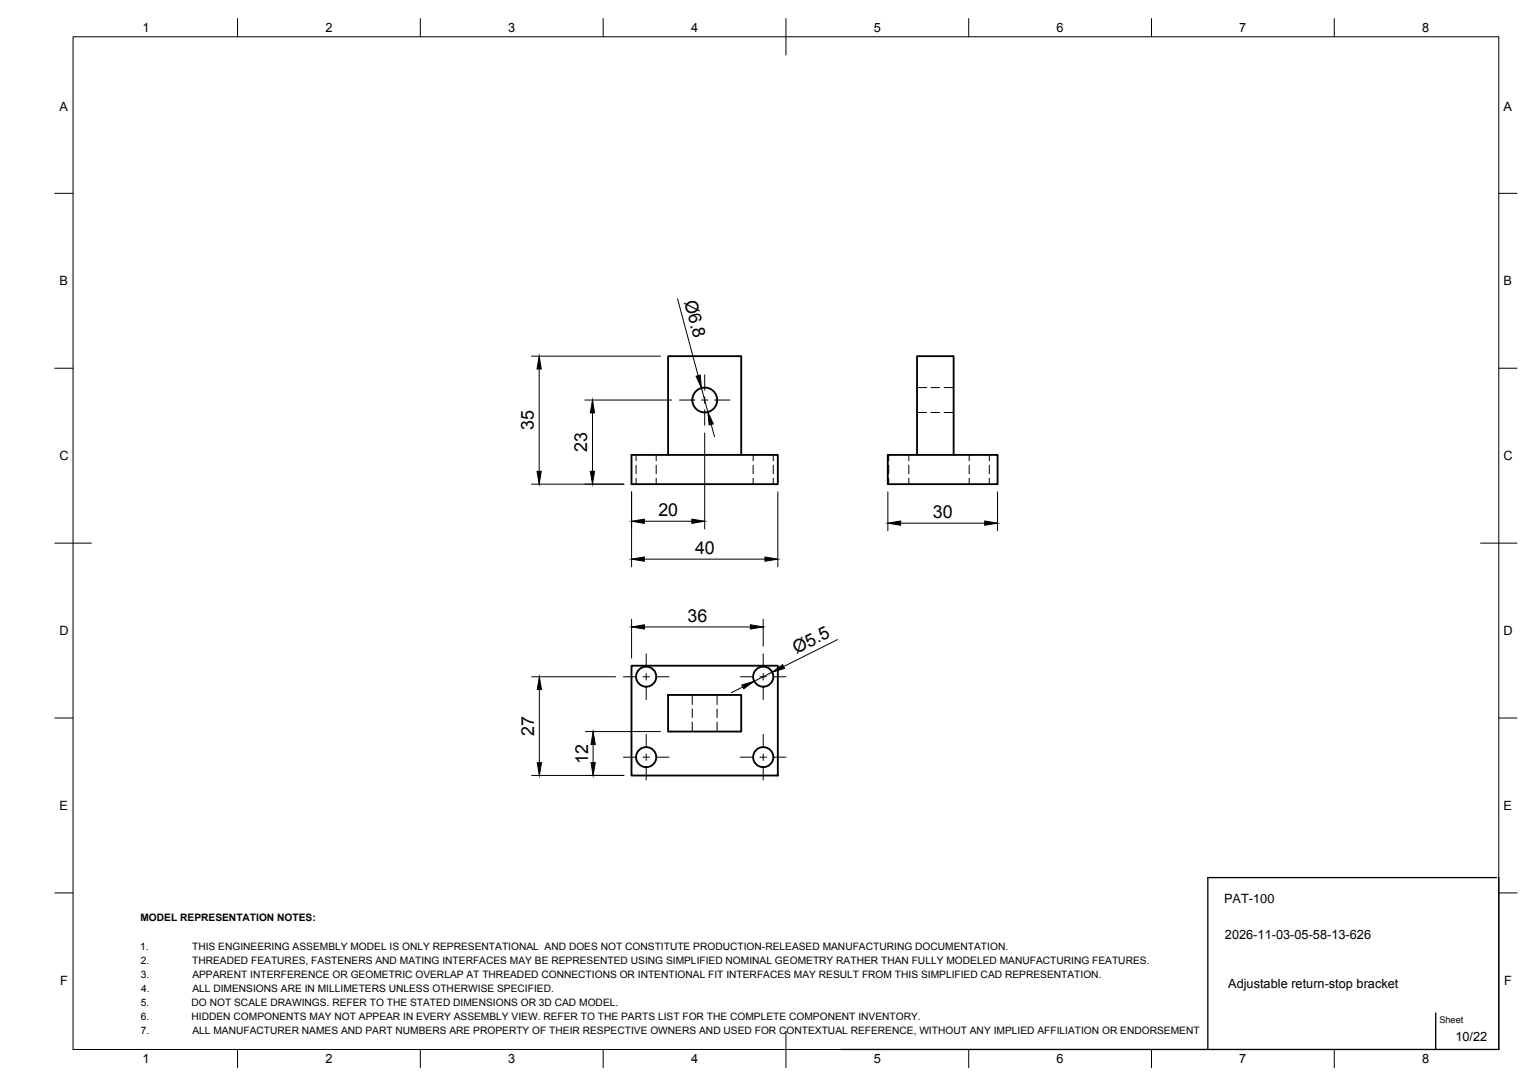
ISO-10303-21;
HEADER;
/* Generated by software containing ST-Developer
 * from STEP Tools, Inc. (www.steptools.com) 
 */

FILE_DESCRIPTION(
/* description */ (''),
/* implementation_level */ '2;1');

FILE_NAME(
/* name */ 'Adjustable return-stop bracket.step',
/* time_stamp */ '2026-10-29T16:43:51-07:00',
/* author */ (''),
/* organization */ (''),
/* preprocessor_version */ 'ST-DEVELOPER v20.2',
/* originating_system */ 'Autodesk Translation Framework v15.17.0.0',
/* authorisation */ '');

FILE_SCHEMA (('AUTOMOTIVE_DESIGN { 1 0 10303 214 3 1 1 }'));
ENDSEC;

DATA;
#10=MECHANICAL_DESIGN_GEOMETRIC_PRESENTATION_REPRESENTATION('',(#371),#10292);
#325=SHAPE_REPRESENTATION_RELATIONSHIP('SRR','None',#10421,#348);
#348=ADVANCED_BREP_SHAPE_REPRESENTATION('',(#393),#10273);
#371=STYLED_ITEM('',(#10607),#393);
#393=MANIFOLD_SOLID_BREP('Body1',#5014);
#455=FACE_BOUND('',#1140,.T.);
#456=FACE_BOUND('',#1142,.T.);
#457=FACE_BOUND('',#1148,.T.);
#458=FACE_BOUND('',#1149,.T.);
#459=FACE_BOUND('',#1150,.T.);
#460=FACE_BOUND('',#1151,.T.);
#461=FACE_BOUND('',#1152,.T.);
#462=FACE_BOUND('',#1154,.T.);
#463=FACE_BOUND('',#1155,.T.);
#464=FACE_BOUND('',#1156,.T.);
#465=FACE_BOUND('',#1157,.T.);
#580=PLANE('',#5462);
#581=PLANE('',#5463);
#582=PLANE('',#5464);
#583=PLANE('',#5465);
#584=PLANE('',#5466);
#585=PLANE('',#5467);
#586=PLANE('',#5468);
#587=PLANE('',#5469);
#588=PLANE('',#5470);
#589=PLANE('',#5471);
#590=PLANE('',#5472);
#794=FACE_OUTER_BOUND('',#1131,.T.);
#795=FACE_OUTER_BOUND('',#1132,.T.);
#796=FACE_OUTER_BOUND('',#1133,.T.);
#797=FACE_OUTER_BOUND('',#1134,.T.);
#798=FACE_OUTER_BOUND('',#1135,.T.);
#799=FACE_OUTER_BOUND('',#1136,.T.);
#800=FACE_OUTER_BOUND('',#1137,.T.);
#801=FACE_OUTER_BOUND('',#1138,.T.);
#802=FACE_OUTER_BOUND('',#1139,.T.);
#803=FACE_OUTER_BOUND('',#1141,.T.);
#804=FACE_OUTER_BOUND('',#1143,.T.);
#805=FACE_OUTER_BOUND('',#1144,.T.);
#806=FACE_OUTER_BOUND('',#1145,.T.);
#807=FACE_OUTER_BOUND('',#1146,.T.);
#808=FACE_OUTER_BOUND('',#1147,.T.);
#809=FACE_OUTER_BOUND('',#1153,.T.);
#1131=EDGE_LOOP('',(#3801,#3802,#3803,#3804));
#1132=EDGE_LOOP('',(#3805,#3806,#3807,#3808));
#1133=EDGE_LOOP('',(#3809,#3810,#3811,#3812));
#1134=EDGE_LOOP('',(#3813,#3814,#3815,#3816));
#1135=EDGE_LOOP('',(#3817,#3818,#3819,#3820));
#1136=EDGE_LOOP('',(#3821,#3822,#3823,#3824));
#1137=EDGE_LOOP('',(#3825,#3826,#3827,#3828));
#1138=EDGE_LOOP('',(#3829,#3830,#3831,#3832));
#1139=EDGE_LOOP('',(#3833,#3834,#3835,#3836));
#1140=EDGE_LOOP('',(#3837));
#1141=EDGE_LOOP('',(#3838,#3839,#3840,#3841));
#1142=EDGE_LOOP('',(#3842));
#1143=EDGE_LOOP('',(#3843,#3844,#3845,#3846));
#1144=EDGE_LOOP('',(#3847,#3848,#3849,#3850));
#1145=EDGE_LOOP('',(#3851,#3852,#3853,#3854));
#1146=EDGE_LOOP('',(#3855,#3856,#3857,#3858));
#1147=EDGE_LOOP('',(#3859,#3860,#3861,#3862));
#1148=EDGE_LOOP('',(#3863,#3864,#3865,#3866));
#1149=EDGE_LOOP('',(#3867));
#1150=EDGE_LOOP('',(#3868));
#1151=EDGE_LOOP('',(#3869));
#1152=EDGE_LOOP('',(#3870));
#1153=EDGE_LOOP('',(#3871,#3872,#3873,#3874));
#1154=EDGE_LOOP('',(#3875));
#1155=EDGE_LOOP('',(#3876));
#1156=EDGE_LOOP('',(#3877));
#1157=EDGE_LOOP('',(#3878));
#1542=LINE('',#7828,#1934);
#1543=LINE('',#7834,#1935);
#1544=LINE('',#7840,#1936);
#1545=LINE('',#7846,#1937);
#1546=LINE('',#7852,#1938);
#1547=LINE('',#7857,#1939);
#1548=LINE('',#7859,#1940);
#1549=LINE('',#7861,#1941);
#1550=LINE('',#7862,#1942);
#1551=LINE('',#7865,#1943);
#1552=LINE('',#7867,#1944);
#1553=LINE('',#7868,#1945);
#1554=LINE('',#7871,#1946);
#1555=LINE('',#7873,#1947);
#1556=LINE('',#7874,#1948);
#1557=LINE('',#7876,#1949);
#1558=LINE('',#7878,#1950);
#1559=LINE('',#7882,#1951);
#1560=LINE('',#7884,#1952);
#1561=LINE('',#7886,#1953);
#1562=LINE('',#7887,#1954);
#1563=LINE('',#7890,#1955);
#1564=LINE('',#7892,#1956);
#1565=LINE('',#7893,#1957);
#1566=LINE('',#7896,#1958);
#1567=LINE('',#7898,#1959);
#1568=LINE('',#7899,#1960);
#1569=LINE('',#7901,#1961);
#1570=LINE('',#7902,#1962);
#1934=VECTOR('',#6315,0.34);
#1935=VECTOR('',#6322,0.275);
#1936=VECTOR('',#6329,0.275);
#1937=VECTOR('',#6336,0.275);
#1938=VECTOR('',#6343,0.275);
#1939=VECTOR('',#6348,1.);
#1940=VECTOR('',#6349,1.);
#1941=VECTOR('',#6350,1.);
#1942=VECTOR('',#6351,1.);
#1943=VECTOR('',#6354,1.);
#1944=VECTOR('',#6355,1.);
#1945=VECTOR('',#6356,1.);
#1946=VECTOR('',#6359,1.);
#1947=VECTOR('',#6360,1.);
#1948=VECTOR('',#6361,1.);
#1949=VECTOR('',#6364,1.);
#1950=VECTOR('',#6367,1.);
#1951=VECTOR('',#6370,1.);
#1952=VECTOR('',#6371,1.);
#1953=VECTOR('',#6372,1.);
#1954=VECTOR('',#6373,1.);
#1955=VECTOR('',#6376,1.);
#1956=VECTOR('',#6377,1.);
#1957=VECTOR('',#6378,1.);
#1958=VECTOR('',#6381,1.);
#1959=VECTOR('',#6382,1.);
#1960=VECTOR('',#6383,1.);
#1961=VECTOR('',#6386,1.);
#1962=VECTOR('',#6387,1.);
#2260=CIRCLE('',#5448,0.34);
#2261=CIRCLE('',#5449,0.34);
#2262=CIRCLE('',#5451,0.275);
#2263=CIRCLE('',#5452,0.275);
#2264=CIRCLE('',#5454,0.275);
#2265=CIRCLE('',#5455,0.275);
#2266=CIRCLE('',#5457,0.275);
#2267=CIRCLE('',#5458,0.275);
#2268=CIRCLE('',#5460,0.275);
#2269=CIRCLE('',#5461,0.275);
#2523=VERTEX_POINT('',#7825);
#2524=VERTEX_POINT('',#7827);
#2525=VERTEX_POINT('',#7831);
#2526=VERTEX_POINT('',#7833);
#2527=VERTEX_POINT('',#7837);
#2528=VERTEX_POINT('',#7839);
#2529=VERTEX_POINT('',#7843);
#2530=VERTEX_POINT('',#7845);
#2531=VERTEX_POINT('',#7849);
#2532=VERTEX_POINT('',#7851);
#2533=VERTEX_POINT('',#7855);
#2534=VERTEX_POINT('',#7856);
#2535=VERTEX_POINT('',#7858);
#2536=VERTEX_POINT('',#7860);
#2537=VERTEX_POINT('',#7864);
#2538=VERTEX_POINT('',#7866);
#2539=VERTEX_POINT('',#7870);
#2540=VERTEX_POINT('',#7872);
#2541=VERTEX_POINT('',#7880);
#2542=VERTEX_POINT('',#7881);
#2543=VERTEX_POINT('',#7883);
#2544=VERTEX_POINT('',#7885);
#2545=VERTEX_POINT('',#7889);
#2546=VERTEX_POINT('',#7891);
#2547=VERTEX_POINT('',#7895);
#2548=VERTEX_POINT('',#7897);
#2991=EDGE_CURVE('',#2523,#2523,#2260,.T.);
#2992=EDGE_CURVE('',#2523,#2524,#1542,.T.);
#2993=EDGE_CURVE('',#2524,#2524,#2261,.T.);
#2994=EDGE_CURVE('',#2525,#2525,#2262,.T.);
#2995=EDGE_CURVE('',#2525,#2526,#1543,.T.);
#2996=EDGE_CURVE('',#2526,#2526,#2263,.T.);
#2997=EDGE_CURVE('',#2527,#2527,#2264,.T.);
#2998=EDGE_CURVE('',#2527,#2528,#1544,.T.);
#2999=EDGE_CURVE('',#2528,#2528,#2265,.T.);
#3000=EDGE_CURVE('',#2529,#2529,#2266,.T.);
#3001=EDGE_CURVE('',#2529,#2530,#1545,.T.);
#3002=EDGE_CURVE('',#2530,#2530,#2267,.T.);
#3003=EDGE_CURVE('',#2531,#2531,#2268,.T.);
#3004=EDGE_CURVE('',#2531,#2532,#1546,.T.);
#3005=EDGE_CURVE('',#2532,#2532,#2269,.T.);
#3006=EDGE_CURVE('',#2533,#2534,#1547,.T.);
#3007=EDGE_CURVE('',#2534,#2535,#1548,.T.);
#3008=EDGE_CURVE('',#2536,#2535,#1549,.T.);
#3009=EDGE_CURVE('',#2533,#2536,#1550,.T.);
#3010=EDGE_CURVE('',#2537,#2533,#1551,.T.);
#3011=EDGE_CURVE('',#2538,#2536,#1552,.T.);
#3012=EDGE_CURVE('',#2537,#2538,#1553,.T.);
#3013=EDGE_CURVE('',#2534,#2539,#1554,.T.);
#3014=EDGE_CURVE('',#2540,#2539,#1555,.T.);
#3015=EDGE_CURVE('',#2535,#2540,#1556,.T.);
#3016=EDGE_CURVE('',#2538,#2540,#1557,.T.);
#3017=EDGE_CURVE('',#2539,#2537,#1558,.T.);
#3018=EDGE_CURVE('',#2541,#2542,#1559,.T.);
#3019=EDGE_CURVE('',#2542,#2543,#1560,.T.);
#3020=EDGE_CURVE('',#2544,#2543,#1561,.T.);
#3021=EDGE_CURVE('',#2541,#2544,#1562,.T.);
#3022=EDGE_CURVE('',#2545,#2541,#1563,.T.);
#3023=EDGE_CURVE('',#2546,#2544,#1564,.T.);
#3024=EDGE_CURVE('',#2545,#2546,#1565,.T.);
#3025=EDGE_CURVE('',#2547,#2545,#1566,.T.);
#3026=EDGE_CURVE('',#2548,#2546,#1567,.T.);
#3027=EDGE_CURVE('',#2547,#2548,#1568,.T.);
#3028=EDGE_CURVE('',#2542,#2547,#1569,.T.);
#3029=EDGE_CURVE('',#2543,#2548,#1570,.T.);
#3801=ORIENTED_EDGE('',*,*,#2991,.F.);
#3802=ORIENTED_EDGE('',*,*,#2992,.T.);
#3803=ORIENTED_EDGE('',*,*,#2993,.F.);
#3804=ORIENTED_EDGE('',*,*,#2992,.F.);
#3805=ORIENTED_EDGE('',*,*,#2994,.F.);
#3806=ORIENTED_EDGE('',*,*,#2995,.T.);
#3807=ORIENTED_EDGE('',*,*,#2996,.F.);
#3808=ORIENTED_EDGE('',*,*,#2995,.F.);
#3809=ORIENTED_EDGE('',*,*,#2997,.F.);
#3810=ORIENTED_EDGE('',*,*,#2998,.T.);
#3811=ORIENTED_EDGE('',*,*,#2999,.F.);
#3812=ORIENTED_EDGE('',*,*,#2998,.F.);
#3813=ORIENTED_EDGE('',*,*,#3000,.F.);
#3814=ORIENTED_EDGE('',*,*,#3001,.T.);
#3815=ORIENTED_EDGE('',*,*,#3002,.F.);
#3816=ORIENTED_EDGE('',*,*,#3001,.F.);
#3817=ORIENTED_EDGE('',*,*,#3003,.F.);
#3818=ORIENTED_EDGE('',*,*,#3004,.T.);
#3819=ORIENTED_EDGE('',*,*,#3005,.F.);
#3820=ORIENTED_EDGE('',*,*,#3004,.F.);
#3821=ORIENTED_EDGE('',*,*,#3006,.T.);
#3822=ORIENTED_EDGE('',*,*,#3007,.T.);
#3823=ORIENTED_EDGE('',*,*,#3008,.F.);
#3824=ORIENTED_EDGE('',*,*,#3009,.F.);
#3825=ORIENTED_EDGE('',*,*,#3010,.T.);
#3826=ORIENTED_EDGE('',*,*,#3009,.T.);
#3827=ORIENTED_EDGE('',*,*,#3011,.F.);
#3828=ORIENTED_EDGE('',*,*,#3012,.F.);
#3829=ORIENTED_EDGE('',*,*,#3013,.T.);
#3830=ORIENTED_EDGE('',*,*,#3014,.F.);
#3831=ORIENTED_EDGE('',*,*,#3015,.F.);
#3832=ORIENTED_EDGE('',*,*,#3007,.F.);
#3833=ORIENTED_EDGE('',*,*,#3015,.T.);
#3834=ORIENTED_EDGE('',*,*,#3016,.F.);
#3835=ORIENTED_EDGE('',*,*,#3011,.T.);
#3836=ORIENTED_EDGE('',*,*,#3008,.T.);
#3837=ORIENTED_EDGE('',*,*,#2993,.T.);
#3838=ORIENTED_EDGE('',*,*,#3013,.F.);
#3839=ORIENTED_EDGE('',*,*,#3006,.F.);
#3840=ORIENTED_EDGE('',*,*,#3010,.F.);
#3841=ORIENTED_EDGE('',*,*,#3017,.F.);
#3842=ORIENTED_EDGE('',*,*,#2991,.T.);
#3843=ORIENTED_EDGE('',*,*,#3018,.T.);
#3844=ORIENTED_EDGE('',*,*,#3019,.T.);
#3845=ORIENTED_EDGE('',*,*,#3020,.F.);
#3846=ORIENTED_EDGE('',*,*,#3021,.F.);
#3847=ORIENTED_EDGE('',*,*,#3022,.T.);
#3848=ORIENTED_EDGE('',*,*,#3021,.T.);
#3849=ORIENTED_EDGE('',*,*,#3023,.F.);
#3850=ORIENTED_EDGE('',*,*,#3024,.F.);
#3851=ORIENTED_EDGE('',*,*,#3025,.T.);
#3852=ORIENTED_EDGE('',*,*,#3024,.T.);
#3853=ORIENTED_EDGE('',*,*,#3026,.F.);
#3854=ORIENTED_EDGE('',*,*,#3027,.F.);
#3855=ORIENTED_EDGE('',*,*,#3028,.T.);
#3856=ORIENTED_EDGE('',*,*,#3027,.T.);
#3857=ORIENTED_EDGE('',*,*,#3029,.F.);
#3858=ORIENTED_EDGE('',*,*,#3019,.F.);
#3859=ORIENTED_EDGE('',*,*,#3029,.T.);
#3860=ORIENTED_EDGE('',*,*,#3026,.T.);
#3861=ORIENTED_EDGE('',*,*,#3023,.T.);
#3862=ORIENTED_EDGE('',*,*,#3020,.T.);
#3863=ORIENTED_EDGE('',*,*,#3014,.T.);
#3864=ORIENTED_EDGE('',*,*,#3017,.T.);
#3865=ORIENTED_EDGE('',*,*,#3012,.T.);
#3866=ORIENTED_EDGE('',*,*,#3016,.T.);
#3867=ORIENTED_EDGE('',*,*,#3005,.T.);
#3868=ORIENTED_EDGE('',*,*,#3002,.T.);
#3869=ORIENTED_EDGE('',*,*,#2999,.T.);
#3870=ORIENTED_EDGE('',*,*,#2996,.T.);
#3871=ORIENTED_EDGE('',*,*,#3028,.F.);
#3872=ORIENTED_EDGE('',*,*,#3018,.F.);
#3873=ORIENTED_EDGE('',*,*,#3022,.F.);
#3874=ORIENTED_EDGE('',*,*,#3025,.F.);
#3875=ORIENTED_EDGE('',*,*,#2994,.T.);
#3876=ORIENTED_EDGE('',*,*,#2997,.T.);
#3877=ORIENTED_EDGE('',*,*,#3000,.T.);
#3878=ORIENTED_EDGE('',*,*,#3003,.T.);
#4667=CYLINDRICAL_SURFACE('',#5447,0.34);
#4668=CYLINDRICAL_SURFACE('',#5450,0.275);
#4669=CYLINDRICAL_SURFACE('',#5453,0.275);
#4670=CYLINDRICAL_SURFACE('',#5456,0.275);
#4671=CYLINDRICAL_SURFACE('',#5459,0.275);
#4803=ADVANCED_FACE('',(#794),#4667,.F.);
#4804=ADVANCED_FACE('',(#795),#4668,.F.);
#4805=ADVANCED_FACE('',(#796),#4669,.F.);
#4806=ADVANCED_FACE('',(#797),#4670,.F.);
#4807=ADVANCED_FACE('',(#798),#4671,.F.);
#4808=ADVANCED_FACE('',(#799),#580,.T.);
#4809=ADVANCED_FACE('',(#800),#581,.T.);
#4810=ADVANCED_FACE('',(#801),#582,.T.);
#4811=ADVANCED_FACE('',(#802,#455),#583,.T.);
#4812=ADVANCED_FACE('',(#803,#456),#584,.F.);
#4813=ADVANCED_FACE('',(#804),#585,.T.);
#4814=ADVANCED_FACE('',(#805),#586,.T.);
#4815=ADVANCED_FACE('',(#806),#587,.T.);
#4816=ADVANCED_FACE('',(#807),#588,.T.);
#4817=ADVANCED_FACE('',(#808,#457,#458,#459,#460,#461),#589,.T.);
#4818=ADVANCED_FACE('',(#809,#462,#463,#464,#465),#590,.F.);
#5014=CLOSED_SHELL('',(#4803,#4804,#4805,#4806,#4807,#4808,#4809,#4810,
#4811,#4812,#4813,#4814,#4815,#4816,#4817,#4818));
#5446=AXIS2_PLACEMENT_3D('',#7823,#6309,#6310);
#5447=AXIS2_PLACEMENT_3D('',#7824,#6311,#6312);
#5448=AXIS2_PLACEMENT_3D('',#7826,#6313,#6314);
#5449=AXIS2_PLACEMENT_3D('',#7829,#6316,#6317);
#5450=AXIS2_PLACEMENT_3D('',#7830,#6318,#6319);
#5451=AXIS2_PLACEMENT_3D('',#7832,#6320,#6321);
#5452=AXIS2_PLACEMENT_3D('',#7835,#6323,#6324);
#5453=AXIS2_PLACEMENT_3D('',#7836,#6325,#6326);
#5454=AXIS2_PLACEMENT_3D('',#7838,#6327,#6328);
#5455=AXIS2_PLACEMENT_3D('',#7841,#6330,#6331);
#5456=AXIS2_PLACEMENT_3D('',#7842,#6332,#6333);
#5457=AXIS2_PLACEMENT_3D('',#7844,#6334,#6335);
#5458=AXIS2_PLACEMENT_3D('',#7847,#6337,#6338);
#5459=AXIS2_PLACEMENT_3D('',#7848,#6339,#6340);
#5460=AXIS2_PLACEMENT_3D('',#7850,#6341,#6342);
#5461=AXIS2_PLACEMENT_3D('',#7853,#6344,#6345);
#5462=AXIS2_PLACEMENT_3D('',#7854,#6346,#6347);
#5463=AXIS2_PLACEMENT_3D('',#7863,#6352,#6353);
#5464=AXIS2_PLACEMENT_3D('',#7869,#6357,#6358);
#5465=AXIS2_PLACEMENT_3D('',#7875,#6362,#6363);
#5466=AXIS2_PLACEMENT_3D('',#7877,#6365,#6366);
#5467=AXIS2_PLACEMENT_3D('',#7879,#6368,#6369);
#5468=AXIS2_PLACEMENT_3D('',#7888,#6374,#6375);
#5469=AXIS2_PLACEMENT_3D('',#7894,#6379,#6380);
#5470=AXIS2_PLACEMENT_3D('',#7900,#6384,#6385);
#5471=AXIS2_PLACEMENT_3D('',#7903,#6388,#6389);
#5472=AXIS2_PLACEMENT_3D('',#7904,#6390,#6391);
#6309=DIRECTION('axis',(0.,0.,1.));
#6310=DIRECTION('refdir',(1.,0.,0.));
#6311=DIRECTION('center_axis',(1.,0.,0.));
#6312=DIRECTION('ref_axis',(0.,0.,-1.));
#6313=DIRECTION('center_axis',(1.,0.,0.));
#6314=DIRECTION('ref_axis',(0.,0.,-1.));
#6315=DIRECTION('',(1.,0.,0.));
#6316=DIRECTION('center_axis',(-1.,0.,0.));
#6317=DIRECTION('ref_axis',(0.,0.,-1.));
#6318=DIRECTION('center_axis',(0.,0.,1.));
#6319=DIRECTION('ref_axis',(1.,0.,0.));
#6320=DIRECTION('center_axis',(0.,0.,1.));
#6321=DIRECTION('ref_axis',(1.,0.,0.));
#6322=DIRECTION('',(0.,0.,1.));
#6323=DIRECTION('center_axis',(0.,0.,-1.));
#6324=DIRECTION('ref_axis',(1.,0.,0.));
#6325=DIRECTION('center_axis',(0.,0.,1.));
#6326=DIRECTION('ref_axis',(1.,0.,0.));
#6327=DIRECTION('center_axis',(0.,0.,1.));
#6328=DIRECTION('ref_axis',(1.,0.,0.));
#6329=DIRECTION('',(0.,0.,1.));
#6330=DIRECTION('center_axis',(0.,0.,-1.));
#6331=DIRECTION('ref_axis',(1.,0.,0.));
#6332=DIRECTION('center_axis',(0.,0.,1.));
#6333=DIRECTION('ref_axis',(1.,0.,0.));
#6334=DIRECTION('center_axis',(0.,0.,1.));
#6335=DIRECTION('ref_axis',(1.,0.,0.));
#6336=DIRECTION('',(0.,0.,1.));
#6337=DIRECTION('center_axis',(0.,0.,-1.));
#6338=DIRECTION('ref_axis',(1.,0.,0.));
#6339=DIRECTION('center_axis',(0.,0.,1.));
#6340=DIRECTION('ref_axis',(1.,0.,0.));
#6341=DIRECTION('center_axis',(0.,0.,1.));
#6342=DIRECTION('ref_axis',(1.,0.,0.));
#6343=DIRECTION('',(0.,0.,1.));
#6344=DIRECTION('center_axis',(0.,0.,-1.));
#6345=DIRECTION('ref_axis',(1.,0.,0.));
#6346=DIRECTION('center_axis',(0.,0.,1.));
#6347=DIRECTION('ref_axis',(0.,-1.,0.));
#6348=DIRECTION('',(0.,-1.,0.));
#6349=DIRECTION('',(1.,0.,0.));
#6350=DIRECTION('',(0.,-1.,0.));
#6351=DIRECTION('',(1.,0.,0.));
#6352=DIRECTION('center_axis',(0.,1.,0.));
#6353=DIRECTION('ref_axis',(0.,0.,1.));
#6354=DIRECTION('',(0.,0.,1.));
#6355=DIRECTION('',(0.,0.,1.));
#6356=DIRECTION('',(1.,0.,0.));
#6357=DIRECTION('center_axis',(0.,-1.,0.));
#6358=DIRECTION('ref_axis',(0.,0.,-1.));
#6359=DIRECTION('',(0.,0.,-1.));
#6360=DIRECTION('',(-1.,0.,0.));
#6361=DIRECTION('',(0.,0.,-1.));
#6362=DIRECTION('center_axis',(1.,0.,0.));
#6363=DIRECTION('ref_axis',(0.,0.,-1.));
#6364=DIRECTION('',(0.,-1.,0.));
#6365=DIRECTION('center_axis',(1.,0.,0.));
#6366=DIRECTION('ref_axis',(0.,0.,-1.));
#6367=DIRECTION('',(0.,1.,0.));
#6368=DIRECTION('center_axis',(0.,1.,0.));
#6369=DIRECTION('ref_axis',(-1.,0.,0.));
#6370=DIRECTION('',(-1.,0.,0.));
#6371=DIRECTION('',(0.,0.,1.));
#6372=DIRECTION('',(-1.,0.,0.));
#6373=DIRECTION('',(0.,0.,1.));
#6374=DIRECTION('center_axis',(1.,0.,0.));
#6375=DIRECTION('ref_axis',(0.,1.,0.));
#6376=DIRECTION('',(0.,1.,0.));
#6377=DIRECTION('',(0.,1.,0.));
#6378=DIRECTION('',(0.,0.,1.));
#6379=DIRECTION('center_axis',(0.,-1.,0.));
#6380=DIRECTION('ref_axis',(1.,0.,0.));
#6381=DIRECTION('',(1.,0.,0.));
#6382=DIRECTION('',(1.,0.,0.));
#6383=DIRECTION('',(0.,0.,1.));
#6384=DIRECTION('center_axis',(-1.,0.,0.));
#6385=DIRECTION('ref_axis',(0.,-1.,0.));
#6386=DIRECTION('',(0.,-1.,0.));
#6387=DIRECTION('',(0.,-1.,0.));
#6388=DIRECTION('center_axis',(0.,0.,1.));
#6389=DIRECTION('ref_axis',(1.,0.,0.));
#6390=DIRECTION('center_axis',(0.,0.,1.));
#6391=DIRECTION('ref_axis',(1.,0.,0.));
#7823=CARTESIAN_POINT('',(0.,0.,0.));
#7824=CARTESIAN_POINT('Origin',(10.1,0.,3.3));
#7825=CARTESIAN_POINT('',(10.2,-4.163799117101E-17,3.64));
#7826=CARTESIAN_POINT('Origin',(10.2,0.,3.3));
#7827=CARTESIAN_POINT('',(11.2,4.163799117101E-17,3.64));
#7828=CARTESIAN_POINT('',(10.1,-4.163799117101E-17,3.64));
#7829=CARTESIAN_POINT('Origin',(11.2,0.,3.3));
#7830=CARTESIAN_POINT('Origin',(11.7,-1.6,0.9));
#7831=CARTESIAN_POINT('',(11.425,-1.6,1.));
#7832=CARTESIAN_POINT('Origin',(11.7,-1.6,1.));
#7833=CARTESIAN_POINT('',(11.425,-1.6,1.8));
#7834=CARTESIAN_POINT('',(11.425,-1.6,0.9));
#7835=CARTESIAN_POINT('Origin',(11.7,-1.6,1.8));
#7836=CARTESIAN_POINT('Origin',(9.5,1.6,0.9));
#7837=CARTESIAN_POINT('',(9.225,1.6,1.));
#7838=CARTESIAN_POINT('Origin',(9.5,1.6,1.));
#7839=CARTESIAN_POINT('',(9.225,1.6,1.8));
#7840=CARTESIAN_POINT('',(9.225,1.6,0.9));
#7841=CARTESIAN_POINT('Origin',(9.5,1.6,1.8));
#7842=CARTESIAN_POINT('Origin',(9.5,-1.6,0.9));
#7843=CARTESIAN_POINT('',(9.225,-1.6,1.));
#7844=CARTESIAN_POINT('Origin',(9.5,-1.6,1.));
#7845=CARTESIAN_POINT('',(9.225,-1.6,1.8));
#7846=CARTESIAN_POINT('',(9.225,-1.6,0.9));
#7847=CARTESIAN_POINT('Origin',(9.5,-1.6,1.8));
#7848=CARTESIAN_POINT('Origin',(11.7,1.6,0.9));
#7849=CARTESIAN_POINT('',(11.425,1.6,1.));
#7850=CARTESIAN_POINT('Origin',(11.7,1.6,1.));
#7851=CARTESIAN_POINT('',(11.425,1.6,1.8));
#7852=CARTESIAN_POINT('',(11.425,1.6,0.9));
#7853=CARTESIAN_POINT('Origin',(11.7,1.6,1.8));
#7854=CARTESIAN_POINT('Origin',(10.2,1.,4.5));
#7855=CARTESIAN_POINT('',(10.2,1.,4.5));
#7856=CARTESIAN_POINT('',(10.2,-1.,4.5));
#7857=CARTESIAN_POINT('',(10.2,1.,4.5));
#7858=CARTESIAN_POINT('',(11.2,-1.,4.5));
#7859=CARTESIAN_POINT('',(10.2,-1.,4.5));
#7860=CARTESIAN_POINT('',(11.2,1.,4.5));
#7861=CARTESIAN_POINT('',(11.2,1.,4.5));
#7862=CARTESIAN_POINT('',(10.2,1.,4.5));
#7863=CARTESIAN_POINT('Origin',(10.2,1.,1.8));
#7864=CARTESIAN_POINT('',(10.2,1.,1.8));
#7865=CARTESIAN_POINT('',(10.2,1.,1.8));
#7866=CARTESIAN_POINT('',(11.2,1.,1.8));
#7867=CARTESIAN_POINT('',(11.2,1.,1.8));
#7868=CARTESIAN_POINT('',(10.35,1.,1.8));
#7869=CARTESIAN_POINT('Origin',(10.2,-1.,4.5));
#7870=CARTESIAN_POINT('',(10.2,-1.,1.8));
#7871=CARTESIAN_POINT('',(10.2,-1.,4.5));
#7872=CARTESIAN_POINT('',(11.2,-1.,1.8));
#7873=CARTESIAN_POINT('',(10.35,-1.,1.8));
#7874=CARTESIAN_POINT('',(11.2,-1.,4.5));
#7875=CARTESIAN_POINT('Origin',(11.2,0.,3.15));
#7876=CARTESIAN_POINT('',(11.2,0.,1.8));
#7877=CARTESIAN_POINT('Origin',(10.2,0.,3.15));
#7878=CARTESIAN_POINT('',(10.2,0.,1.8));
#7879=CARTESIAN_POINT('Origin',(12.,2.,1.));
#7880=CARTESIAN_POINT('',(12.,2.,1.));
#7881=CARTESIAN_POINT('',(9.,2.,1.));
#7882=CARTESIAN_POINT('',(12.,2.,1.));
#7883=CARTESIAN_POINT('',(9.,2.,1.8));
#7884=CARTESIAN_POINT('',(9.,2.,1.));
#7885=CARTESIAN_POINT('',(12.,2.,1.8));
#7886=CARTESIAN_POINT('',(12.,2.,1.8));
#7887=CARTESIAN_POINT('',(12.,2.,1.));
#7888=CARTESIAN_POINT('Origin',(12.,-2.,1.));
#7889=CARTESIAN_POINT('',(12.,-2.,1.));
#7890=CARTESIAN_POINT('',(12.,-2.,1.));
#7891=CARTESIAN_POINT('',(12.,-2.,1.8));
#7892=CARTESIAN_POINT('',(12.,-2.,1.8));
#7893=CARTESIAN_POINT('',(12.,-2.,1.));
#7894=CARTESIAN_POINT('Origin',(9.,-2.,1.));
#7895=CARTESIAN_POINT('',(9.,-2.,1.));
#7896=CARTESIAN_POINT('',(9.,-2.,1.));
#7897=CARTESIAN_POINT('',(9.,-2.,1.8));
#7898=CARTESIAN_POINT('',(9.,-2.,1.8));
#7899=CARTESIAN_POINT('',(9.,-2.,1.));
#7900=CARTESIAN_POINT('Origin',(9.,2.,1.));
#7901=CARTESIAN_POINT('',(9.,2.,1.));
#7902=CARTESIAN_POINT('',(9.,2.,1.8));
#7903=CARTESIAN_POINT('Origin',(10.5,0.,1.8));
#7904=CARTESIAN_POINT('Origin',(10.5,0.,1.));
#10245=UNCERTAINTY_MEASURE_WITH_UNIT(LENGTH_MEASURE(0.001),#10293,
'DISTANCE_ACCURACY_VALUE',
'Maximum model space distance between geometric entities at asserted c
onnectivities');
#10264=UNCERTAINTY_MEASURE_WITH_UNIT(LENGTH_MEASURE(0.001),#10293,
'DISTANCE_ACCURACY_VALUE',
'Maximum model space distance between geometric entities at asserted c
onnectivities');
#10273=(
GEOMETRIC_REPRESENTATION_CONTEXT(3)
GLOBAL_UNCERTAINTY_ASSIGNED_CONTEXT((#10245))
GLOBAL_UNIT_ASSIGNED_CONTEXT((#10293,#10295,#10296))
REPRESENTATION_CONTEXT('','3D')
);
#10292=(
GEOMETRIC_REPRESENTATION_CONTEXT(3)
GLOBAL_UNCERTAINTY_ASSIGNED_CONTEXT((#10264))
GLOBAL_UNIT_ASSIGNED_CONTEXT((#10293,#10295,#10296))
REPRESENTATION_CONTEXT('','3D')
);
#10293=(
LENGTH_UNIT()
NAMED_UNIT(*)
SI_UNIT(.CENTI.,.METRE.)
);
#10295=(
NAMED_UNIT(*)
PLANE_ANGLE_UNIT()
SI_UNIT($,.RADIAN.)
);
#10296=(
NAMED_UNIT(*)
SI_UNIT($,.STERADIAN.)
SOLID_ANGLE_UNIT()
);
#10305=SHAPE_DEFINITION_REPRESENTATION(#10332,#10421);
#10332=PRODUCT_DEFINITION_SHAPE('',$,#10449);
#10421=SHAPE_REPRESENTATION('',(#5446),#10273);
#10440=PRODUCT_DEFINITION_CONTEXT('part definition',#10523,'design');
#10449=PRODUCT_DEFINITION('Adjustable return-stop bracket',
'Adjustable return-stop bracket',#10476,#10440);
#10476=PRODUCT_DEFINITION_FORMATION('',$,#10533);
#10523=APPLICATION_CONTEXT(
'Core Data for Automotive Mechanical Design Process');
#10524=PRODUCT_CONTEXT('part definition',#10523,'mechanical');
#10533=PRODUCT('Adjustable return-stop bracket',
'Adjustable return-stop bracket','Adjustable return-stop bracket',(#10524));
#10601=COLOUR_RGB('Dark Blue',0.08,0.2,0.34);
#10602=FILL_AREA_STYLE_COLOUR('',#10601);
#10603=FILL_AREA_STYLE('',(#10602));
#10604=SURFACE_STYLE_FILL_AREA(#10603);
#10605=SURFACE_SIDE_STYLE('',(#10604));
#10606=SURFACE_STYLE_USAGE(.BOTH.,#10605);
#10607=PRESENTATION_STYLE_ASSIGNMENT((#10606));
ENDSEC;
END-ISO-10303-21;
